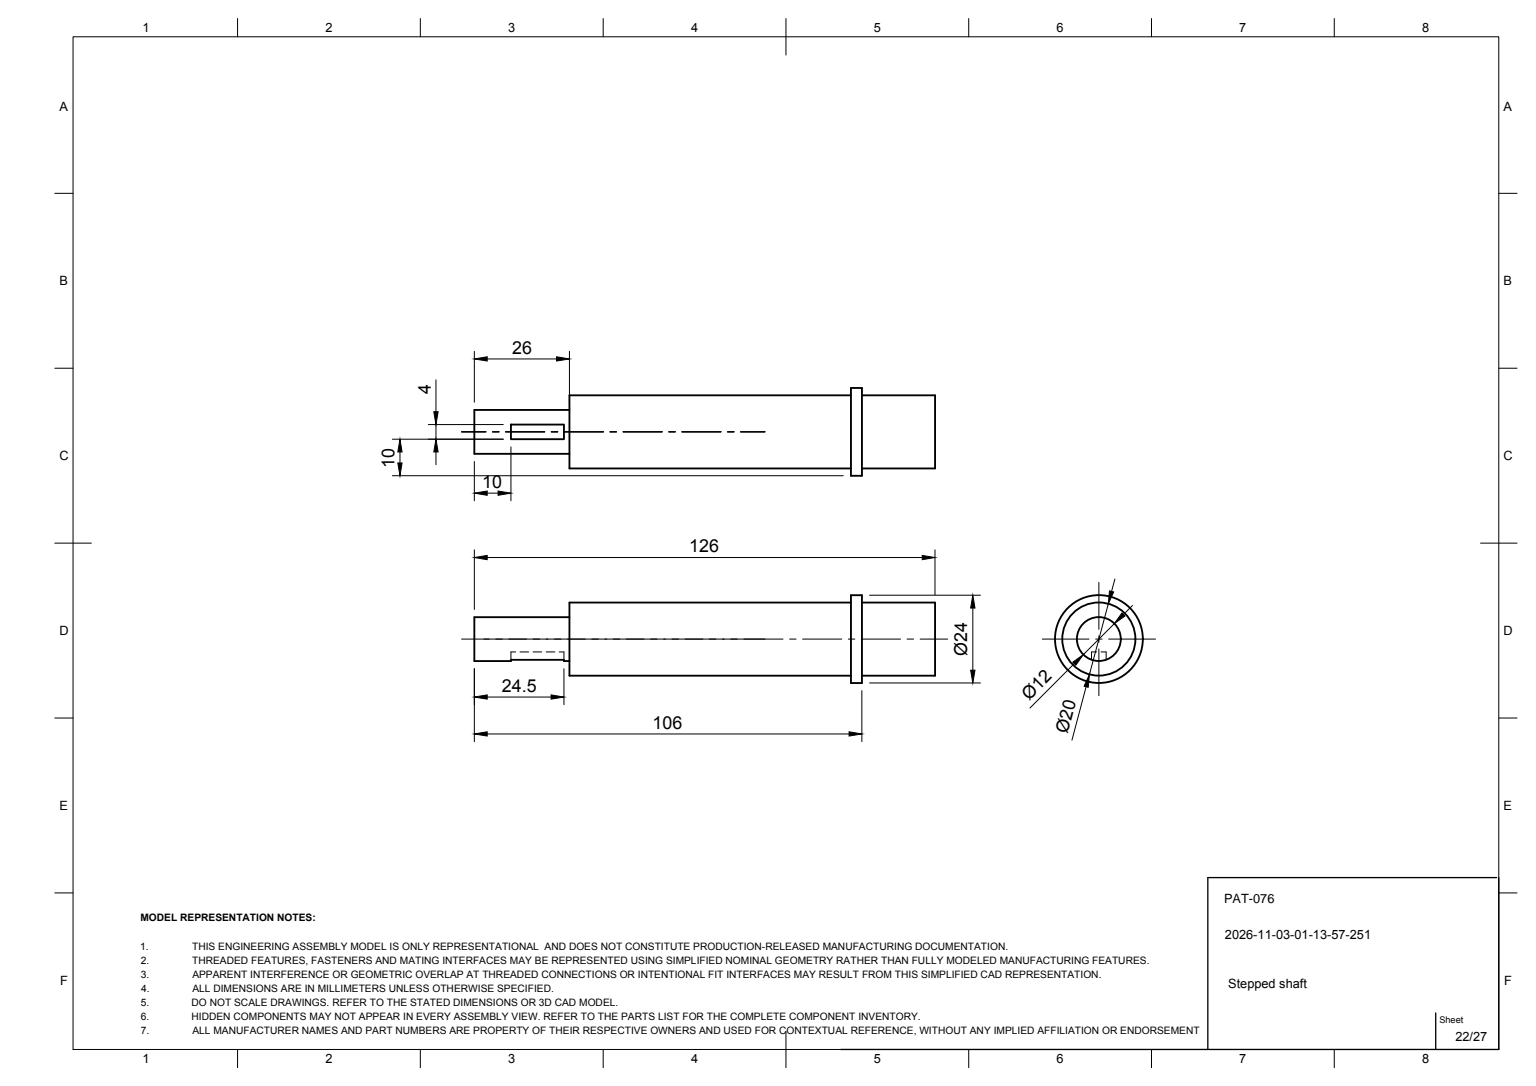
ISO-10303-21;
HEADER;
/* Generated by software containing ST-Developer
 * from STEP Tools, Inc. (www.steptools.com) 
 */

FILE_DESCRIPTION(
/* description */ ('Overhung pulley bearing cartridge'),
/* implementation_level */ '2;1');

FILE_NAME(
/* name */ 'Stepped shaft.step',
/* time_stamp */ '2026-10-28T03:22:33-07:00',
/* author */ (''),
/* organization */ (''),
/* preprocessor_version */ 'ST-DEVELOPER v20.2',
/* originating_system */ 'Autodesk Translation Framework v15.17.0.0',
/* authorisation */ '');

FILE_SCHEMA (('AUTOMOTIVE_DESIGN { 1 0 10303 214 3 1 1 }'));
ENDSEC;

DATA;
#10=MECHANICAL_DESIGN_GEOMETRIC_PRESENTATION_REPRESENTATION('',(#306),#10963);
#254=SHAPE_REPRESENTATION_RELATIONSHIP('SRR','None',#11076,#276);
#276=ADVANCED_BREP_SHAPE_REPRESENTATION('',(#334),#10956);
#306=STYLED_ITEM('',(#11253),#334);
#334=MANIFOLD_SOLID_BREP('Body1',#5675);
#407=FACE_BOUND('',#1157,.T.);
#408=FACE_BOUND('',#1160,.T.);
#409=FACE_BOUND('',#1162,.T.);
#410=FACE_BOUND('',#1167,.T.);
#530=PLANE('',#6321);
#531=PLANE('',#6322);
#532=PLANE('',#6324);
#533=PLANE('',#6325);
#534=PLANE('',#6326);
#535=PLANE('',#6331);
#536=PLANE('',#6332);
#537=PLANE('',#6335);
#538=PLANE('',#6343);
#539=PLANE('',#6344);
#756=FACE_OUTER_BOUND('',#1151,.T.);
#757=FACE_OUTER_BOUND('',#1152,.T.);
#758=FACE_OUTER_BOUND('',#1153,.T.);
#759=FACE_OUTER_BOUND('',#1154,.T.);
#760=FACE_OUTER_BOUND('',#1155,.T.);
#761=FACE_OUTER_BOUND('',#1156,.T.);
#762=FACE_OUTER_BOUND('',#1158,.T.);
#763=FACE_OUTER_BOUND('',#1159,.T.);
#764=FACE_OUTER_BOUND('',#1161,.T.);
#765=FACE_OUTER_BOUND('',#1163,.T.);
#766=FACE_OUTER_BOUND('',#1164,.T.);
#767=FACE_OUTER_BOUND('',#1165,.T.);
#768=FACE_OUTER_BOUND('',#1166,.T.);
#769=FACE_OUTER_BOUND('',#1168,.T.);
#1151=EDGE_LOOP('',(#4375,#4376,#4377,#4378));
#1152=EDGE_LOOP('',(#4379,#4380,#4381,#4382));
#1153=EDGE_LOOP('',(#4383,#4384,#4385,#4386));
#1154=EDGE_LOOP('',(#4387,#4388,#4389,#4390));
#1155=EDGE_LOOP('',(#4391,#4392,#4393,#4394));
#1156=EDGE_LOOP('',(#4395,#4396,#4397,#4398));
#1157=EDGE_LOOP('',(#4399,#4400,#4401,#4402));
#1158=EDGE_LOOP('',(#4403));
#1159=EDGE_LOOP('',(#4404));
#1160=EDGE_LOOP('',(#4405));
#1161=EDGE_LOOP('',(#4406));
#1162=EDGE_LOOP('',(#4407));
#1163=EDGE_LOOP('',(#4408,#4409,#4410,#4411));
#1164=EDGE_LOOP('',(#4412,#4413,#4414,#4415));
#1165=EDGE_LOOP('',(#4416,#4417,#4418,#4419));
#1166=EDGE_LOOP('',(#4420));
#1167=EDGE_LOOP('',(#4421));
#1168=EDGE_LOOP('',(#4422));
#1501=LINE('',#9730,#1843);
#1502=LINE('',#9732,#1844);
#1503=LINE('',#9734,#1845);
#1504=LINE('',#9735,#1846);
#1505=LINE('',#9740,#1847);
#1506=LINE('',#9741,#1848);
#1507=LINE('',#9744,#1849);
#1508=LINE('',#9746,#1850);
#1509=LINE('',#9747,#1851);
#1510=LINE('',#9749,#1852);
#1511=LINE('',#9756,#1853);
#1512=LINE('',#9770,#1854);
#1513=LINE('',#9773,#1855);
#1514=LINE('',#9778,#1856);
#1843=VECTOR('',#7655,1.);
#1844=VECTOR('',#7656,1.);
#1845=VECTOR('',#7657,1.);
#1846=VECTOR('',#7658,1.);
#1847=VECTOR('',#7663,1.);
#1848=VECTOR('',#7664,1.);
#1849=VECTOR('',#7667,1.);
#1850=VECTOR('',#7668,1.);
#1851=VECTOR('',#7669,1.);
#1852=VECTOR('',#7672,1.);
#1853=VECTOR('',#7681,0.6);
#1854=VECTOR('',#7700,1.2);
#1855=VECTOR('',#7703,1.);
#1856=VECTOR('',#7710,1.);
#2182=CIRCLE('',#6323,0.6);
#2183=CIRCLE('',#6327,0.6);
#2184=CIRCLE('',#6329,0.6);
#2185=CIRCLE('',#6330,0.6);
#2186=CIRCLE('',#6333,1.2);
#2187=CIRCLE('',#6334,1.);
#2188=CIRCLE('',#6336,1.2);
#2189=CIRCLE('',#6337,1.);
#2190=CIRCLE('',#6340,1.);
#2191=CIRCLE('',#6342,1.);
#2629=VERTEX_POINT('',#9728);
#2630=VERTEX_POINT('',#9729);
#2631=VERTEX_POINT('',#9731);
#2632=VERTEX_POINT('',#9733);
#2633=VERTEX_POINT('',#9737);
#2634=VERTEX_POINT('',#9739);
#2635=VERTEX_POINT('',#9743);
#2636=VERTEX_POINT('',#9745);
#2637=VERTEX_POINT('',#9753);
#2638=VERTEX_POINT('',#9755);
#2639=VERTEX_POINT('',#9760);
#2640=VERTEX_POINT('',#9762);
#2641=VERTEX_POINT('',#9765);
#2642=VERTEX_POINT('',#9767);
#2643=VERTEX_POINT('',#9772);
#2644=VERTEX_POINT('',#9776);
#3257=EDGE_CURVE('',#2629,#2630,#1501,.T.);
#3258=EDGE_CURVE('',#2629,#2631,#1502,.T.);
#3259=EDGE_CURVE('',#2632,#2631,#1503,.T.);
#3260=EDGE_CURVE('',#2632,#2630,#1504,.T.);
#3261=EDGE_CURVE('',#2630,#2633,#2182,.T.);
#3262=EDGE_CURVE('',#2634,#2632,#1505,.T.);
#3263=EDGE_CURVE('',#2633,#2634,#1506,.T.);
#3264=EDGE_CURVE('',#2633,#2635,#1507,.T.);
#3265=EDGE_CURVE('',#2634,#2636,#1508,.T.);
#3266=EDGE_CURVE('',#2636,#2635,#1509,.T.);
#3267=EDGE_CURVE('',#2631,#2636,#1510,.T.);
#3268=EDGE_CURVE('',#2635,#2629,#2183,.T.);
#3269=EDGE_CURVE('',#2637,#2637,#2184,.T.);
#3270=EDGE_CURVE('',#2637,#2638,#1511,.T.);
#3271=EDGE_CURVE('',#2638,#2638,#2185,.T.);
#3272=EDGE_CURVE('',#2639,#2639,#2186,.T.);
#3273=EDGE_CURVE('',#2640,#2640,#2187,.T.);
#3274=EDGE_CURVE('',#2641,#2641,#2188,.T.);
#3275=EDGE_CURVE('',#2642,#2642,#2189,.T.);
#3276=EDGE_CURVE('',#2639,#2641,#1512,.T.);
#3277=EDGE_CURVE('',#2642,#2643,#1513,.T.);
#3278=EDGE_CURVE('',#2643,#2643,#2190,.T.);
#3279=EDGE_CURVE('',#2644,#2644,#2191,.T.);
#3280=EDGE_CURVE('',#2644,#2640,#1514,.T.);
#4375=ORIENTED_EDGE('',*,*,#3257,.F.);
#4376=ORIENTED_EDGE('',*,*,#3258,.T.);
#4377=ORIENTED_EDGE('',*,*,#3259,.F.);
#4378=ORIENTED_EDGE('',*,*,#3260,.T.);
#4379=ORIENTED_EDGE('',*,*,#3261,.F.);
#4380=ORIENTED_EDGE('',*,*,#3260,.F.);
#4381=ORIENTED_EDGE('',*,*,#3262,.F.);
#4382=ORIENTED_EDGE('',*,*,#3263,.F.);
#4383=ORIENTED_EDGE('',*,*,#3264,.F.);
#4384=ORIENTED_EDGE('',*,*,#3263,.T.);
#4385=ORIENTED_EDGE('',*,*,#3265,.T.);
#4386=ORIENTED_EDGE('',*,*,#3266,.T.);
#4387=ORIENTED_EDGE('',*,*,#3262,.T.);
#4388=ORIENTED_EDGE('',*,*,#3259,.T.);
#4389=ORIENTED_EDGE('',*,*,#3267,.T.);
#4390=ORIENTED_EDGE('',*,*,#3265,.F.);
#4391=ORIENTED_EDGE('',*,*,#3268,.F.);
#4392=ORIENTED_EDGE('',*,*,#3266,.F.);
#4393=ORIENTED_EDGE('',*,*,#3267,.F.);
#4394=ORIENTED_EDGE('',*,*,#3258,.F.);
#4395=ORIENTED_EDGE('',*,*,#3269,.F.);
#4396=ORIENTED_EDGE('',*,*,#3270,.T.);
#4397=ORIENTED_EDGE('',*,*,#3271,.F.);
#4398=ORIENTED_EDGE('',*,*,#3270,.F.);
#4399=ORIENTED_EDGE('',*,*,#3264,.T.);
#4400=ORIENTED_EDGE('',*,*,#3268,.T.);
#4401=ORIENTED_EDGE('',*,*,#3257,.T.);
#4402=ORIENTED_EDGE('',*,*,#3261,.T.);
#4403=ORIENTED_EDGE('',*,*,#3269,.T.);
#4404=ORIENTED_EDGE('',*,*,#3272,.T.);
#4405=ORIENTED_EDGE('',*,*,#3273,.F.);
#4406=ORIENTED_EDGE('',*,*,#3274,.F.);
#4407=ORIENTED_EDGE('',*,*,#3275,.F.);
#4408=ORIENTED_EDGE('',*,*,#3272,.F.);
#4409=ORIENTED_EDGE('',*,*,#3276,.T.);
#4410=ORIENTED_EDGE('',*,*,#3274,.T.);
#4411=ORIENTED_EDGE('',*,*,#3276,.F.);
#4412=ORIENTED_EDGE('',*,*,#3275,.T.);
#4413=ORIENTED_EDGE('',*,*,#3277,.T.);
#4414=ORIENTED_EDGE('',*,*,#3278,.T.);
#4415=ORIENTED_EDGE('',*,*,#3277,.F.);
#4416=ORIENTED_EDGE('',*,*,#3279,.F.);
#4417=ORIENTED_EDGE('',*,*,#3280,.T.);
#4418=ORIENTED_EDGE('',*,*,#3273,.T.);
#4419=ORIENTED_EDGE('',*,*,#3280,.F.);
#4420=ORIENTED_EDGE('',*,*,#3279,.T.);
#4421=ORIENTED_EDGE('',*,*,#3271,.T.);
#4422=ORIENTED_EDGE('',*,*,#3278,.F.);
#5220=CYLINDRICAL_SURFACE('',#6328,0.6);
#5221=CYLINDRICAL_SURFACE('',#6338,1.2);
#5222=CYLINDRICAL_SURFACE('',#6339,1.);
#5223=CYLINDRICAL_SURFACE('',#6341,1.);
#5500=ADVANCED_FACE('',(#756),#530,.F.);
#5501=ADVANCED_FACE('',(#757),#531,.T.);
#5502=ADVANCED_FACE('',(#758),#532,.F.);
#5503=ADVANCED_FACE('',(#759),#533,.F.);
#5504=ADVANCED_FACE('',(#760),#534,.F.);
#5505=ADVANCED_FACE('',(#761,#407),#5220,.T.);
#5506=ADVANCED_FACE('',(#762),#535,.T.);
#5507=ADVANCED_FACE('',(#763,#408),#536,.T.);
#5508=ADVANCED_FACE('',(#764,#409),#537,.F.);
#5509=ADVANCED_FACE('',(#765),#5221,.T.);
#5510=ADVANCED_FACE('',(#766),#5222,.T.);
#5511=ADVANCED_FACE('',(#767),#5223,.T.);
#5512=ADVANCED_FACE('',(#768,#410),#538,.T.);
#5513=ADVANCED_FACE('',(#769),#539,.F.);
#5675=CLOSED_SHELL('',(#5500,#5501,#5502,#5503,#5504,#5505,#5506,#5507,
#5508,#5509,#5510,#5511,#5512,#5513));
#6320=AXIS2_PLACEMENT_3D('',#9726,#7651,#7652);
#6321=AXIS2_PLACEMENT_3D('',#9727,#7653,#7654);
#6322=AXIS2_PLACEMENT_3D('',#9736,#7659,#7660);
#6323=AXIS2_PLACEMENT_3D('',#9738,#7661,#7662);
#6324=AXIS2_PLACEMENT_3D('',#9742,#7665,#7666);
#6325=AXIS2_PLACEMENT_3D('',#9748,#7670,#7671);
#6326=AXIS2_PLACEMENT_3D('',#9750,#7673,#7674);
#6327=AXIS2_PLACEMENT_3D('',#9751,#7675,#7676);
#6328=AXIS2_PLACEMENT_3D('',#9752,#7677,#7678);
#6329=AXIS2_PLACEMENT_3D('',#9754,#7679,#7680);
#6330=AXIS2_PLACEMENT_3D('',#9757,#7682,#7683);
#6331=AXIS2_PLACEMENT_3D('',#9758,#7684,#7685);
#6332=AXIS2_PLACEMENT_3D('',#9759,#7686,#7687);
#6333=AXIS2_PLACEMENT_3D('',#9761,#7688,#7689);
#6334=AXIS2_PLACEMENT_3D('',#9763,#7690,#7691);
#6335=AXIS2_PLACEMENT_3D('',#9764,#7692,#7693);
#6336=AXIS2_PLACEMENT_3D('',#9766,#7694,#7695);
#6337=AXIS2_PLACEMENT_3D('',#9768,#7696,#7697);
#6338=AXIS2_PLACEMENT_3D('',#9769,#7698,#7699);
#6339=AXIS2_PLACEMENT_3D('',#9771,#7701,#7702);
#6340=AXIS2_PLACEMENT_3D('',#9774,#7704,#7705);
#6341=AXIS2_PLACEMENT_3D('',#9775,#7706,#7707);
#6342=AXIS2_PLACEMENT_3D('',#9777,#7708,#7709);
#6343=AXIS2_PLACEMENT_3D('',#9779,#7711,#7712);
#6344=AXIS2_PLACEMENT_3D('',#9780,#7713,#7714);
#7651=DIRECTION('axis',(0.,0.,1.));
#7652=DIRECTION('refdir',(1.,0.,0.));
#7653=DIRECTION('center_axis',(-1.,0.,0.));
#7654=DIRECTION('ref_axis',(0.,0.,1.));
#7655=DIRECTION('',(0.,-1.,0.));
#7656=DIRECTION('',(0.,0.,1.));
#7657=DIRECTION('',(0.,1.,0.));
#7658=DIRECTION('',(0.,0.,-1.));
#7659=DIRECTION('center_axis',(0.,1.,0.));
#7660=DIRECTION('ref_axis',(1.,0.,0.));
#7661=DIRECTION('center_axis',(0.,-1.,0.));
#7662=DIRECTION('ref_axis',(1.,0.,0.));
#7663=DIRECTION('',(-1.,0.,0.));
#7664=DIRECTION('',(0.,0.,1.));
#7665=DIRECTION('center_axis',(1.,0.,0.));
#7666=DIRECTION('ref_axis',(0.,0.,-1.));
#7667=DIRECTION('',(0.,1.,0.));
#7668=DIRECTION('',(0.,1.,0.));
#7669=DIRECTION('',(0.,0.,-1.));
#7670=DIRECTION('center_axis',(0.,0.,1.));
#7671=DIRECTION('ref_axis',(1.,0.,0.));
#7672=DIRECTION('',(1.,0.,0.));
#7673=DIRECTION('center_axis',(0.,1.,0.));
#7674=DIRECTION('ref_axis',(0.,0.,1.));
#7675=DIRECTION('center_axis',(0.,1.,0.));
#7676=DIRECTION('ref_axis',(1.,0.,0.));
#7677=DIRECTION('center_axis',(0.,1.,0.));
#7678=DIRECTION('ref_axis',(1.,0.,0.));
#7679=DIRECTION('center_axis',(0.,1.,0.));
#7680=DIRECTION('ref_axis',(1.,0.,0.));
#7681=DIRECTION('',(0.,-1.,0.));
#7682=DIRECTION('center_axis',(0.,-1.,0.));
#7683=DIRECTION('ref_axis',(1.,0.,0.));
#7684=DIRECTION('center_axis',(0.,1.,0.));
#7685=DIRECTION('ref_axis',(1.,0.,0.));
#7686=DIRECTION('center_axis',(0.,1.,0.));
#7687=DIRECTION('ref_axis',(1.,0.,0.));
#7688=DIRECTION('center_axis',(0.,1.,0.));
#7689=DIRECTION('ref_axis',(1.,0.,0.));
#7690=DIRECTION('center_axis',(0.,1.,0.));
#7691=DIRECTION('ref_axis',(1.,0.,0.));
#7692=DIRECTION('center_axis',(0.,1.,0.));
#7693=DIRECTION('ref_axis',(1.,0.,0.));
#7694=DIRECTION('center_axis',(0.,1.,0.));
#7695=DIRECTION('ref_axis',(1.,0.,0.));
#7696=DIRECTION('center_axis',(0.,-1.,0.));
#7697=DIRECTION('ref_axis',(1.,0.,0.));
#7698=DIRECTION('center_axis',(0.,1.,0.));
#7699=DIRECTION('ref_axis',(1.,0.,0.));
#7700=DIRECTION('',(0.,-1.,0.));
#7701=DIRECTION('center_axis',(0.,1.,0.));
#7702=DIRECTION('ref_axis',(1.,0.,0.));
#7703=DIRECTION('',(0.,-1.,0.));
#7704=DIRECTION('center_axis',(0.,1.,0.));
#7705=DIRECTION('ref_axis',(1.,0.,0.));
#7706=DIRECTION('center_axis',(0.,1.,0.));
#7707=DIRECTION('ref_axis',(1.,0.,0.));
#7708=DIRECTION('center_axis',(0.,1.,0.));
#7709=DIRECTION('ref_axis',(1.,0.,0.));
#7710=DIRECTION('',(0.,-1.,0.));
#7711=DIRECTION('center_axis',(0.,1.,0.));
#7712=DIRECTION('ref_axis',(1.,0.,0.));
#7713=DIRECTION('center_axis',(0.,1.,0.));
#7714=DIRECTION('ref_axis',(1.,0.,0.));
#9726=CARTESIAN_POINT('',(0.,0.,0.));
#9727=CARTESIAN_POINT('Origin',(-0.2,8.15,3.8));
#9728=CARTESIAN_POINT('',(-0.2,9.6,3.93431457505076));
#9729=CARTESIAN_POINT('',(-0.2,8.15,3.93431457505076));
#9730=CARTESIAN_POINT('',(-0.2,8.,3.93431457505076));
#9731=CARTESIAN_POINT('',(-0.2,9.6,4.15));
#9732=CARTESIAN_POINT('',(-0.2,9.6,4.15));
#9733=CARTESIAN_POINT('',(-0.2,8.15,4.15));
#9734=CARTESIAN_POINT('',(-0.2,8.15,4.15));
#9735=CARTESIAN_POINT('',(-0.2,8.15,4.15));
#9736=CARTESIAN_POINT('Origin',(0.,8.15,3.975));
#9737=CARTESIAN_POINT('',(0.2,8.15,3.93431457505076));
#9738=CARTESIAN_POINT('Origin',(0.,8.15,4.5));
#9739=CARTESIAN_POINT('',(0.2,8.15,4.15));
#9740=CARTESIAN_POINT('',(0.2,8.15,4.15));
#9741=CARTESIAN_POINT('',(0.2,8.15,3.8));
#9742=CARTESIAN_POINT('Origin',(0.2,8.15,4.15));
#9743=CARTESIAN_POINT('',(0.2,9.6,3.93431457505076));
#9744=CARTESIAN_POINT('',(0.2,8.,3.93431457505076));
#9745=CARTESIAN_POINT('',(0.2,9.6,4.15));
#9746=CARTESIAN_POINT('',(0.2,8.15,4.15));
#9747=CARTESIAN_POINT('',(0.2,9.6,3.8));
#9748=CARTESIAN_POINT('Origin',(-0.2,8.15,4.15));
#9749=CARTESIAN_POINT('',(0.2,9.6,4.15));
#9750=CARTESIAN_POINT('Origin',(0.,9.6,3.975));
#9751=CARTESIAN_POINT('Origin',(0.,9.6,4.5));
#9752=CARTESIAN_POINT('Origin',(0.,8.,4.5));
#9753=CARTESIAN_POINT('',(-0.6,10.6,4.5));
#9754=CARTESIAN_POINT('Origin',(0.,10.6,4.5));
#9755=CARTESIAN_POINT('',(-0.6,8.,4.5));
#9756=CARTESIAN_POINT('',(-0.6,8.,4.5));
#9757=CARTESIAN_POINT('Origin',(0.,8.,4.5));
#9758=CARTESIAN_POINT('Origin',(0.,10.6,4.5));
#9759=CARTESIAN_POINT('Origin',(0.,0.3,4.5));
#9760=CARTESIAN_POINT('',(-1.2,0.3,4.5));
#9761=CARTESIAN_POINT('Origin',(0.,0.3,4.5));
#9762=CARTESIAN_POINT('',(-1.,0.3,4.5));
#9763=CARTESIAN_POINT('Origin',(0.,0.3,4.5));
#9764=CARTESIAN_POINT('Origin',(0.,0.,4.5));
#9765=CARTESIAN_POINT('',(-1.2,0.,4.5));
#9766=CARTESIAN_POINT('Origin',(0.,0.,4.5));
#9767=CARTESIAN_POINT('',(-1.,0.,4.5));
#9768=CARTESIAN_POINT('Origin',(0.,0.,4.5));
#9769=CARTESIAN_POINT('Origin',(0.,0.,4.5));
#9770=CARTESIAN_POINT('',(-1.2,0.,4.5));
#9771=CARTESIAN_POINT('Origin',(0.,-2.,4.5));
#9772=CARTESIAN_POINT('',(-1.,-2.,4.5));
#9773=CARTESIAN_POINT('',(-1.,-2.,4.5));
#9774=CARTESIAN_POINT('Origin',(0.,-2.,4.5));
#9775=CARTESIAN_POINT('Origin',(0.,-2.,4.5));
#9776=CARTESIAN_POINT('',(-1.,8.,4.5));
#9777=CARTESIAN_POINT('Origin',(0.,8.,4.5));
#9778=CARTESIAN_POINT('',(-1.,-2.,4.5));
#9779=CARTESIAN_POINT('Origin',(0.,8.,4.5));
#9780=CARTESIAN_POINT('Origin',(0.,-2.,4.5));
#10929=UNCERTAINTY_MEASURE_WITH_UNIT(LENGTH_MEASURE(0.001),#10964,
'DISTANCE_ACCURACY_VALUE',
'Maximum model space distance between geometric entities at asserted c
onnectivities');
#10936=UNCERTAINTY_MEASURE_WITH_UNIT(LENGTH_MEASURE(0.001),#10964,
'DISTANCE_ACCURACY_VALUE',
'Maximum model space distance between geometric entities at asserted c
onnectivities');
#10956=(
GEOMETRIC_REPRESENTATION_CONTEXT(3)
GLOBAL_UNCERTAINTY_ASSIGNED_CONTEXT((#10929))
GLOBAL_UNIT_ASSIGNED_CONTEXT((#10964,#10966,#10967))
REPRESENTATION_CONTEXT('','3D')
);
#10963=(
GEOMETRIC_REPRESENTATION_CONTEXT(3)
GLOBAL_UNCERTAINTY_ASSIGNED_CONTEXT((#10936))
GLOBAL_UNIT_ASSIGNED_CONTEXT((#10964,#10966,#10967))
REPRESENTATION_CONTEXT('','3D')
);
#10964=(
LENGTH_UNIT()
NAMED_UNIT(*)
SI_UNIT(.CENTI.,.METRE.)
);
#10966=(
NAMED_UNIT(*)
PLANE_ANGLE_UNIT()
SI_UNIT($,.RADIAN.)
);
#10967=(
NAMED_UNIT(*)
SI_UNIT($,.STERADIAN.)
SOLID_ANGLE_UNIT()
);
#10987=SHAPE_DEFINITION_REPRESENTATION(#11040,#11076);
#11040=PRODUCT_DEFINITION_SHAPE('',$,#11103);
#11076=SHAPE_REPRESENTATION('',(#6320),#10956);
#11083=PRODUCT_DEFINITION_CONTEXT('part definition',#11163,'design');
#11103=PRODUCT_DEFINITION('Stepped shaft','Stepped shaft',#11129,#11083);
#11129=PRODUCT_DEFINITION_FORMATION('',$,#11184);
#11163=APPLICATION_CONTEXT(
'Core Data for Automotive Mechanical Design Process');
#11164=PRODUCT_CONTEXT('part definition',#11163,'mechanical');
#11184=PRODUCT('Stepped shaft','Stepped shaft','Stepped shaft',(#11164));
#11247=COLOUR_RGB('Grey',0.48,0.52,0.57);
#11248=FILL_AREA_STYLE_COLOUR('',#11247);
#11249=FILL_AREA_STYLE('',(#11248));
#11250=SURFACE_STYLE_FILL_AREA(#11249);
#11251=SURFACE_SIDE_STYLE('',(#11250));
#11252=SURFACE_STYLE_USAGE(.BOTH.,#11251);
#11253=PRESENTATION_STYLE_ASSIGNMENT((#11252));
ENDSEC;
END-ISO-10303-21;
